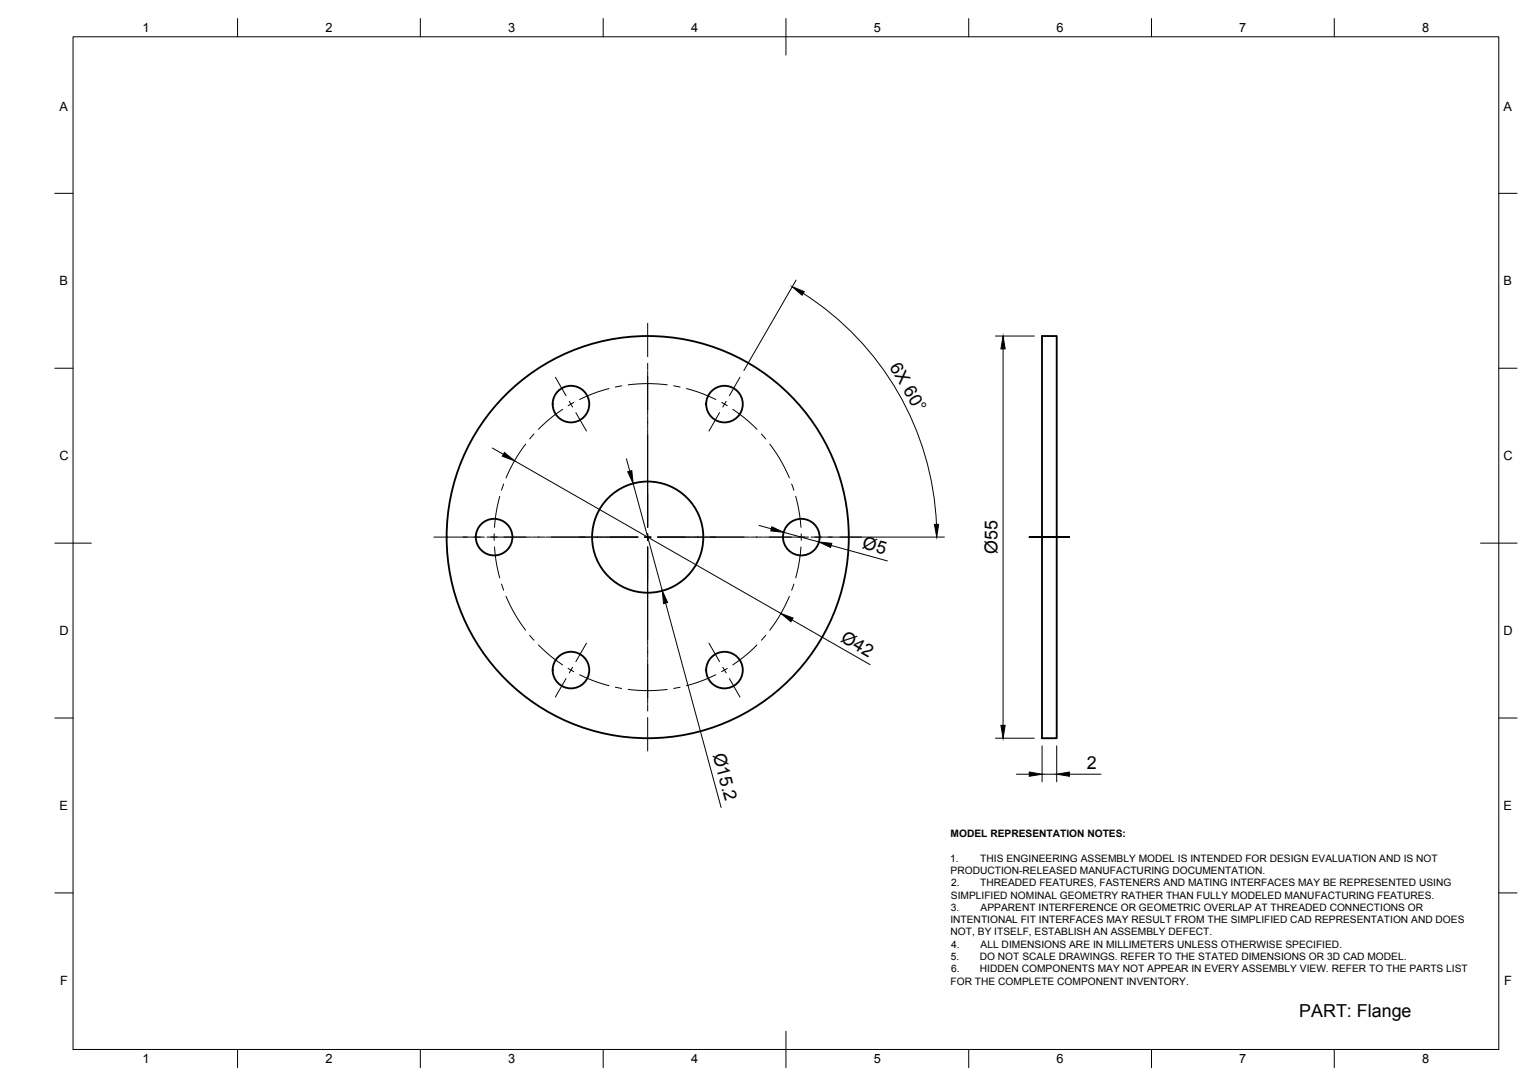
ISO-10303-21;
HEADER;
/* Generated by software containing ST-Developer
 * from STEP Tools, Inc. (www.steptools.com) 
 */

FILE_DESCRIPTION(
/* description */ ('STEP AP214'),
/* implementation_level */ '2;1');

FILE_NAME(
/* name */ 'Flange.step',
/* time_stamp */ '2026-10-05T13:15:56-07:00',
/* author */ (''),
/* organization */ (''),
/* preprocessor_version */ 'ST-DEVELOPER v20.2',
/* originating_system */ 'Autodesk Translation Framework v15.15.0.0',
/* authorisation */ '');

FILE_SCHEMA (('AUTOMOTIVE_DESIGN { 1 0 10303 214 3 1 1 }'));
ENDSEC;

DATA;
#10=MECHANICAL_DESIGN_GEOMETRIC_PRESENTATION_REPRESENTATION('',(#1352),#37881);
#1328=SHAPE_REPRESENTATION_RELATIONSHIP('SRR','None',#37961,#1340);
#1340=ADVANCED_BREP_SHAPE_REPRESENTATION('',(#1364),#37876);
#1352=STYLED_ITEM('',(#38023),#1364);
#1364=MANIFOLD_SOLID_BREP('Body1',#10826);
#1447=FACE_BOUND('',#2815,.T.);
#1448=FACE_BOUND('',#2816,.T.);
#1449=FACE_BOUND('',#2817,.T.);
#1450=FACE_BOUND('',#2818,.T.);
#1451=FACE_BOUND('',#2819,.T.);
#1452=FACE_BOUND('',#2820,.T.);
#1453=FACE_BOUND('',#2821,.T.);
#1454=FACE_BOUND('',#2823,.T.);
#1455=FACE_BOUND('',#2824,.T.);
#1456=FACE_BOUND('',#2825,.T.);
#1457=FACE_BOUND('',#2826,.T.);
#1458=FACE_BOUND('',#2827,.T.);
#1459=FACE_BOUND('',#2828,.T.);
#1460=FACE_BOUND('',#2829,.T.);
#1533=PLANE('',#11792);
#1534=PLANE('',#11793);
#2127=FACE_OUTER_BOUND('',#2806,.T.);
#2128=FACE_OUTER_BOUND('',#2807,.T.);
#2129=FACE_OUTER_BOUND('',#2808,.T.);
#2130=FACE_OUTER_BOUND('',#2809,.T.);
#2131=FACE_OUTER_BOUND('',#2810,.T.);
#2132=FACE_OUTER_BOUND('',#2811,.T.);
#2133=FACE_OUTER_BOUND('',#2812,.T.);
#2134=FACE_OUTER_BOUND('',#2813,.T.);
#2135=FACE_OUTER_BOUND('',#2814,.T.);
#2136=FACE_OUTER_BOUND('',#2822,.T.);
#2806=EDGE_LOOP('',(#9821,#9822,#9823,#9824));
#2807=EDGE_LOOP('',(#9825,#9826,#9827,#9828));
#2808=EDGE_LOOP('',(#9829,#9830,#9831,#9832));
#2809=EDGE_LOOP('',(#9833,#9834,#9835,#9836));
#2810=EDGE_LOOP('',(#9837,#9838,#9839,#9840));
#2811=EDGE_LOOP('',(#9841,#9842,#9843,#9844));
#2812=EDGE_LOOP('',(#9845,#9846,#9847,#9848));
#2813=EDGE_LOOP('',(#9849,#9850,#9851,#9852));
#2814=EDGE_LOOP('',(#9853));
#2815=EDGE_LOOP('',(#9854));
#2816=EDGE_LOOP('',(#9855));
#2817=EDGE_LOOP('',(#9856));
#2818=EDGE_LOOP('',(#9857));
#2819=EDGE_LOOP('',(#9858));
#2820=EDGE_LOOP('',(#9859));
#2821=EDGE_LOOP('',(#9860));
#2822=EDGE_LOOP('',(#9861));
#2823=EDGE_LOOP('',(#9862));
#2824=EDGE_LOOP('',(#9863));
#2825=EDGE_LOOP('',(#9864));
#2826=EDGE_LOOP('',(#9865));
#2827=EDGE_LOOP('',(#9866));
#2828=EDGE_LOOP('',(#9867));
#2829=EDGE_LOOP('',(#9868));
#3098=LINE('',#37593,#3399);
#3099=LINE('',#37599,#3400);
#3100=LINE('',#37605,#3401);
#3101=LINE('',#37611,#3402);
#3102=LINE('',#37617,#3403);
#3103=LINE('',#37623,#3404);
#3104=LINE('',#37629,#3405);
#3105=LINE('',#37635,#3406);
#3399=VECTOR('',#13729,2.5);
#3400=VECTOR('',#13736,2.5);
#3401=VECTOR('',#13743,2.5);
#3402=VECTOR('',#13750,2.5);
#3403=VECTOR('',#13757,2.5);
#3404=VECTOR('',#13764,2.5);
#3405=VECTOR('',#13771,7.6);
#3406=VECTOR('',#13778,27.5);
#3968=CIRCLE('',#11769,2.5);
#3969=CIRCLE('',#11770,2.5);
#3970=CIRCLE('',#11772,2.5);
#3971=CIRCLE('',#11773,2.5);
#3972=CIRCLE('',#11775,2.5);
#3973=CIRCLE('',#11776,2.5);
#3974=CIRCLE('',#11778,2.5);
#3975=CIRCLE('',#11779,2.5);
#3976=CIRCLE('',#11781,2.5);
#3977=CIRCLE('',#11782,2.5);
#3978=CIRCLE('',#11784,2.5);
#3979=CIRCLE('',#11785,2.5);
#3980=CIRCLE('',#11787,7.6);
#3981=CIRCLE('',#11788,7.6);
#3982=CIRCLE('',#11790,27.5);
#3983=CIRCLE('',#11791,27.5);
#5004=VERTEX_POINT('',#37590);
#5005=VERTEX_POINT('',#37592);
#5006=VERTEX_POINT('',#37596);
#5007=VERTEX_POINT('',#37598);
#5008=VERTEX_POINT('',#37602);
#5009=VERTEX_POINT('',#37604);
#5010=VERTEX_POINT('',#37608);
#5011=VERTEX_POINT('',#37610);
#5012=VERTEX_POINT('',#37614);
#5013=VERTEX_POINT('',#37616);
#5014=VERTEX_POINT('',#37620);
#5015=VERTEX_POINT('',#37622);
#5016=VERTEX_POINT('',#37626);
#5017=VERTEX_POINT('',#37628);
#5018=VERTEX_POINT('',#37632);
#5019=VERTEX_POINT('',#37634);
#6621=EDGE_CURVE('',#5004,#5004,#3968,.T.);
#6622=EDGE_CURVE('',#5004,#5005,#3098,.T.);
#6623=EDGE_CURVE('',#5005,#5005,#3969,.T.);
#6624=EDGE_CURVE('',#5006,#5006,#3970,.T.);
#6625=EDGE_CURVE('',#5006,#5007,#3099,.T.);
#6626=EDGE_CURVE('',#5007,#5007,#3971,.T.);
#6627=EDGE_CURVE('',#5008,#5008,#3972,.T.);
#6628=EDGE_CURVE('',#5008,#5009,#3100,.T.);
#6629=EDGE_CURVE('',#5009,#5009,#3973,.T.);
#6630=EDGE_CURVE('',#5010,#5010,#3974,.T.);
#6631=EDGE_CURVE('',#5010,#5011,#3101,.T.);
#6632=EDGE_CURVE('',#5011,#5011,#3975,.T.);
#6633=EDGE_CURVE('',#5012,#5012,#3976,.T.);
#6634=EDGE_CURVE('',#5012,#5013,#3102,.T.);
#6635=EDGE_CURVE('',#5013,#5013,#3977,.T.);
#6636=EDGE_CURVE('',#5014,#5014,#3978,.T.);
#6637=EDGE_CURVE('',#5014,#5015,#3103,.T.);
#6638=EDGE_CURVE('',#5015,#5015,#3979,.T.);
#6639=EDGE_CURVE('',#5016,#5016,#3980,.T.);
#6640=EDGE_CURVE('',#5016,#5017,#3104,.T.);
#6641=EDGE_CURVE('',#5017,#5017,#3981,.T.);
#6642=EDGE_CURVE('',#5018,#5018,#3982,.T.);
#6643=EDGE_CURVE('',#5018,#5019,#3105,.T.);
#6644=EDGE_CURVE('',#5019,#5019,#3983,.T.);
#9821=ORIENTED_EDGE('',*,*,#6621,.T.);
#9822=ORIENTED_EDGE('',*,*,#6622,.T.);
#9823=ORIENTED_EDGE('',*,*,#6623,.F.);
#9824=ORIENTED_EDGE('',*,*,#6622,.F.);
#9825=ORIENTED_EDGE('',*,*,#6624,.T.);
#9826=ORIENTED_EDGE('',*,*,#6625,.T.);
#9827=ORIENTED_EDGE('',*,*,#6626,.F.);
#9828=ORIENTED_EDGE('',*,*,#6625,.F.);
#9829=ORIENTED_EDGE('',*,*,#6627,.T.);
#9830=ORIENTED_EDGE('',*,*,#6628,.T.);
#9831=ORIENTED_EDGE('',*,*,#6629,.F.);
#9832=ORIENTED_EDGE('',*,*,#6628,.F.);
#9833=ORIENTED_EDGE('',*,*,#6630,.T.);
#9834=ORIENTED_EDGE('',*,*,#6631,.T.);
#9835=ORIENTED_EDGE('',*,*,#6632,.F.);
#9836=ORIENTED_EDGE('',*,*,#6631,.F.);
#9837=ORIENTED_EDGE('',*,*,#6633,.T.);
#9838=ORIENTED_EDGE('',*,*,#6634,.T.);
#9839=ORIENTED_EDGE('',*,*,#6635,.F.);
#9840=ORIENTED_EDGE('',*,*,#6634,.F.);
#9841=ORIENTED_EDGE('',*,*,#6636,.T.);
#9842=ORIENTED_EDGE('',*,*,#6637,.T.);
#9843=ORIENTED_EDGE('',*,*,#6638,.F.);
#9844=ORIENTED_EDGE('',*,*,#6637,.F.);
#9845=ORIENTED_EDGE('',*,*,#6639,.T.);
#9846=ORIENTED_EDGE('',*,*,#6640,.T.);
#9847=ORIENTED_EDGE('',*,*,#6641,.F.);
#9848=ORIENTED_EDGE('',*,*,#6640,.F.);
#9849=ORIENTED_EDGE('',*,*,#6642,.T.);
#9850=ORIENTED_EDGE('',*,*,#6643,.T.);
#9851=ORIENTED_EDGE('',*,*,#6644,.F.);
#9852=ORIENTED_EDGE('',*,*,#6643,.F.);
#9853=ORIENTED_EDGE('',*,*,#6644,.T.);
#9854=ORIENTED_EDGE('',*,*,#6639,.F.);
#9855=ORIENTED_EDGE('',*,*,#6633,.F.);
#9856=ORIENTED_EDGE('',*,*,#6627,.F.);
#9857=ORIENTED_EDGE('',*,*,#6621,.F.);
#9858=ORIENTED_EDGE('',*,*,#6624,.F.);
#9859=ORIENTED_EDGE('',*,*,#6630,.F.);
#9860=ORIENTED_EDGE('',*,*,#6636,.F.);
#9861=ORIENTED_EDGE('',*,*,#6642,.F.);
#9862=ORIENTED_EDGE('',*,*,#6641,.T.);
#9863=ORIENTED_EDGE('',*,*,#6638,.T.);
#9864=ORIENTED_EDGE('',*,*,#6635,.T.);
#9865=ORIENTED_EDGE('',*,*,#6632,.T.);
#9866=ORIENTED_EDGE('',*,*,#6629,.T.);
#9867=ORIENTED_EDGE('',*,*,#6626,.T.);
#9868=ORIENTED_EDGE('',*,*,#6623,.T.);
#10197=CYLINDRICAL_SURFACE('',#11768,2.5);
#10198=CYLINDRICAL_SURFACE('',#11771,2.5);
#10199=CYLINDRICAL_SURFACE('',#11774,2.5);
#10200=CYLINDRICAL_SURFACE('',#11777,2.5);
#10201=CYLINDRICAL_SURFACE('',#11780,2.5);
#10202=CYLINDRICAL_SURFACE('',#11783,2.5);
#10203=CYLINDRICAL_SURFACE('',#11786,7.6);
#10204=CYLINDRICAL_SURFACE('',#11789,27.5);
#10772=ADVANCED_FACE('',(#2127),#10197,.F.);
#10773=ADVANCED_FACE('',(#2128),#10198,.F.);
#10774=ADVANCED_FACE('',(#2129),#10199,.F.);
#10775=ADVANCED_FACE('',(#2130),#10200,.F.);
#10776=ADVANCED_FACE('',(#2131),#10201,.F.);
#10777=ADVANCED_FACE('',(#2132),#10202,.F.);
#10778=ADVANCED_FACE('',(#2133),#10203,.F.);
#10779=ADVANCED_FACE('',(#2134),#10204,.T.);
#10780=ADVANCED_FACE('',(#2135,#1447,#1448,#1449,#1450,#1451,#1452,#1453),
#1533,.T.);
#10781=ADVANCED_FACE('',(#2136,#1454,#1455,#1456,#1457,#1458,#1459,#1460),
#1534,.F.);
#10826=CLOSED_SHELL('',(#10772,#10773,#10774,#10775,#10776,#10777,#10778,
#10779,#10780,#10781));
#11767=AXIS2_PLACEMENT_3D('',#37588,#13723,#13724);
#11768=AXIS2_PLACEMENT_3D('',#37589,#13725,#13726);
#11769=AXIS2_PLACEMENT_3D('',#37591,#13727,#13728);
#11770=AXIS2_PLACEMENT_3D('',#37594,#13730,#13731);
#11771=AXIS2_PLACEMENT_3D('',#37595,#13732,#13733);
#11772=AXIS2_PLACEMENT_3D('',#37597,#13734,#13735);
#11773=AXIS2_PLACEMENT_3D('',#37600,#13737,#13738);
#11774=AXIS2_PLACEMENT_3D('',#37601,#13739,#13740);
#11775=AXIS2_PLACEMENT_3D('',#37603,#13741,#13742);
#11776=AXIS2_PLACEMENT_3D('',#37606,#13744,#13745);
#11777=AXIS2_PLACEMENT_3D('',#37607,#13746,#13747);
#11778=AXIS2_PLACEMENT_3D('',#37609,#13748,#13749);
#11779=AXIS2_PLACEMENT_3D('',#37612,#13751,#13752);
#11780=AXIS2_PLACEMENT_3D('',#37613,#13753,#13754);
#11781=AXIS2_PLACEMENT_3D('',#37615,#13755,#13756);
#11782=AXIS2_PLACEMENT_3D('',#37618,#13758,#13759);
#11783=AXIS2_PLACEMENT_3D('',#37619,#13760,#13761);
#11784=AXIS2_PLACEMENT_3D('',#37621,#13762,#13763);
#11785=AXIS2_PLACEMENT_3D('',#37624,#13765,#13766);
#11786=AXIS2_PLACEMENT_3D('',#37625,#13767,#13768);
#11787=AXIS2_PLACEMENT_3D('',#37627,#13769,#13770);
#11788=AXIS2_PLACEMENT_3D('',#37630,#13772,#13773);
#11789=AXIS2_PLACEMENT_3D('',#37631,#13774,#13775);
#11790=AXIS2_PLACEMENT_3D('',#37633,#13776,#13777);
#11791=AXIS2_PLACEMENT_3D('',#37636,#13779,#13780);
#11792=AXIS2_PLACEMENT_3D('',#37637,#13781,#13782);
#11793=AXIS2_PLACEMENT_3D('',#37638,#13783,#13784);
#13723=DIRECTION('axis',(0.,0.,1.));
#13724=DIRECTION('refdir',(1.,0.,0.));
#13725=DIRECTION('center_axis',(-2.36658271566304E-30,1.04667633103075E-31,
-1.));
#13726=DIRECTION('ref_axis',(-1.,-2.47704611391098E-61,2.36658271566304E-30));
#13727=DIRECTION('center_axis',(2.36658271566304E-30,-1.04667633103075E-31,
1.));
#13728=DIRECTION('ref_axis',(1.,2.47704611391098E-61,-2.36658271566304E-30));
#13729=DIRECTION('',(-2.36658271566304E-30,1.04667633103075E-31,-1.));
#13730=DIRECTION('center_axis',(2.36658271566304E-30,-1.04667633103075E-31,
1.));
#13731=DIRECTION('ref_axis',(1.,2.47704611391098E-61,-2.36658271566304E-30));
#13732=DIRECTION('center_axis',(-2.36658271566304E-30,1.04667633103075E-31,
-1.));
#13733=DIRECTION('ref_axis',(-1.,-2.47704611391098E-61,2.36658271566304E-30));
#13734=DIRECTION('center_axis',(2.36658271566304E-30,-1.04667633103075E-31,
1.));
#13735=DIRECTION('ref_axis',(1.,2.47704611391098E-61,-2.36658271566304E-30));
#13736=DIRECTION('',(-2.36658271566304E-30,1.04667633103075E-31,-1.));
#13737=DIRECTION('center_axis',(2.36658271566304E-30,-1.04667633103075E-31,
1.));
#13738=DIRECTION('ref_axis',(1.,2.47704611391098E-61,-2.36658271566304E-30));
#13739=DIRECTION('center_axis',(-2.36658271566304E-30,1.04667633103075E-31,
-1.));
#13740=DIRECTION('ref_axis',(-1.,-2.47704611391098E-61,2.36658271566304E-30));
#13741=DIRECTION('center_axis',(2.36658271566304E-30,-1.04667633103075E-31,
1.));
#13742=DIRECTION('ref_axis',(1.,2.47704611391098E-61,-2.36658271566304E-30));
#13743=DIRECTION('',(-2.36658271566304E-30,1.04667633103075E-31,-1.));
#13744=DIRECTION('center_axis',(2.36658271566304E-30,-1.04667633103075E-31,
1.));
#13745=DIRECTION('ref_axis',(1.,2.47704611391098E-61,-2.36658271566304E-30));
#13746=DIRECTION('center_axis',(-2.36658271566304E-30,1.04667633103075E-31,
-1.));
#13747=DIRECTION('ref_axis',(-1.,-2.47704611391098E-61,2.36658271566304E-30));
#13748=DIRECTION('center_axis',(2.36658271566304E-30,-1.04667633103075E-31,
1.));
#13749=DIRECTION('ref_axis',(1.,2.47704611391098E-61,-2.36658271566304E-30));
#13750=DIRECTION('',(-2.36658271566304E-30,1.04667633103075E-31,-1.));
#13751=DIRECTION('center_axis',(2.36658271566304E-30,-1.04667633103075E-31,
1.));
#13752=DIRECTION('ref_axis',(1.,2.47704611391098E-61,-2.36658271566304E-30));
#13753=DIRECTION('center_axis',(-2.36658271566304E-30,1.04667633103075E-31,
-1.));
#13754=DIRECTION('ref_axis',(-1.,-2.47704611391098E-61,2.36658271566304E-30));
#13755=DIRECTION('center_axis',(2.36658271566304E-30,-1.04667633103075E-31,
1.));
#13756=DIRECTION('ref_axis',(1.,2.47704611391098E-61,-2.36658271566304E-30));
#13757=DIRECTION('',(-2.36658271566304E-30,1.04667633103075E-31,-1.));
#13758=DIRECTION('center_axis',(2.36658271566304E-30,-1.04667633103075E-31,
1.));
#13759=DIRECTION('ref_axis',(1.,2.47704611391098E-61,-2.36658271566304E-30));
#13760=DIRECTION('center_axis',(-2.36658271566304E-30,1.04667633103075E-31,
-1.));
#13761=DIRECTION('ref_axis',(-1.,-2.47704611391098E-61,2.36658271566304E-30));
#13762=DIRECTION('center_axis',(2.36658271566304E-30,-1.04667633103075E-31,
1.));
#13763=DIRECTION('ref_axis',(1.,2.47704611391098E-61,-2.36658271566304E-30));
#13764=DIRECTION('',(-2.36658271566304E-30,1.04667633103075E-31,-1.));
#13765=DIRECTION('center_axis',(2.36658271566304E-30,-1.04667633103075E-31,
1.));
#13766=DIRECTION('ref_axis',(1.,2.47704611391098E-61,-2.36658271566304E-30));
#13767=DIRECTION('center_axis',(-2.36658271566304E-30,1.04667633103075E-31,
-1.));
#13768=DIRECTION('ref_axis',(-1.,-2.47704611391098E-61,2.36658271566304E-30));
#13769=DIRECTION('center_axis',(2.36658271566304E-30,-1.04667633103075E-31,
1.));
#13770=DIRECTION('ref_axis',(1.,2.47704611391098E-61,-2.36658271566304E-30));
#13771=DIRECTION('',(-2.36658271566304E-30,1.04667633103075E-31,-1.));
#13772=DIRECTION('center_axis',(2.36658271566304E-30,-1.04667633103075E-31,
1.));
#13773=DIRECTION('ref_axis',(1.,2.47704611391098E-61,-2.36658271566304E-30));
#13774=DIRECTION('center_axis',(-2.36658271566304E-30,1.04667633103075E-31,
-1.));
#13775=DIRECTION('ref_axis',(-1.,-2.47704611391098E-61,2.36658271566304E-30));
#13776=DIRECTION('center_axis',(2.36658271566304E-30,-1.04667633103075E-31,
1.));
#13777=DIRECTION('ref_axis',(1.,2.47704611391098E-61,-2.36658271566304E-30));
#13778=DIRECTION('',(2.36658271566304E-30,-1.04667633103075E-31,1.));
#13779=DIRECTION('center_axis',(2.36658271566304E-30,-1.04667633103075E-31,
1.));
#13780=DIRECTION('ref_axis',(1.,2.47704611391098E-61,-2.36658271566304E-30));
#13781=DIRECTION('center_axis',(-2.36658271566304E-30,-1.04667633103075E-31,
1.));
#13782=DIRECTION('ref_axis',(1.,0.,2.36658271566304E-30));
#13783=DIRECTION('center_axis',(-2.36658271566304E-30,-1.04667633103075E-31,
1.));
#13784=DIRECTION('ref_axis',(1.,0.,2.36658271566304E-30));
#37588=CARTESIAN_POINT('',(0.,0.,0.));
#37589=CARTESIAN_POINT('Origin',(-18.1865334794732,10.5,1.));
#37590=CARTESIAN_POINT('',(-15.6865334794732,10.5,1.));
#37591=CARTESIAN_POINT('Origin',(-18.1865334794732,10.5,1.));
#37592=CARTESIAN_POINT('',(-15.6865334794732,10.5,-1.));
#37593=CARTESIAN_POINT('',(-15.6865334794732,10.5,1.));
#37594=CARTESIAN_POINT('Origin',(-18.1865334794732,10.5,-1.));
#37595=CARTESIAN_POINT('Origin',(-18.1865334794732,-10.5,1.));
#37596=CARTESIAN_POINT('',(-15.6865334794732,-10.5,1.));
#37597=CARTESIAN_POINT('Origin',(-18.1865334794732,-10.5,1.));
#37598=CARTESIAN_POINT('',(-15.6865334794732,-10.5,-1.));
#37599=CARTESIAN_POINT('',(-15.6865334794732,-10.5,1.));
#37600=CARTESIAN_POINT('Origin',(-18.1865334794732,-10.5,-1.));
#37601=CARTESIAN_POINT('Origin',(6.93889390390723E-15,-21.,1.));
#37602=CARTESIAN_POINT('',(2.50000000000001,-21.,1.));
#37603=CARTESIAN_POINT('Origin',(6.93889390390723E-15,-21.,1.));
#37604=CARTESIAN_POINT('',(2.50000000000001,-21.,-1.));
#37605=CARTESIAN_POINT('',(2.50000000000001,-21.,1.));
#37606=CARTESIAN_POINT('Origin',(6.93889390390723E-15,-21.,-1.));
#37607=CARTESIAN_POINT('Origin',(18.1865334794732,-10.5,1.));
#37608=CARTESIAN_POINT('',(20.6865334794732,-10.5,1.));
#37609=CARTESIAN_POINT('Origin',(18.1865334794732,-10.5,1.));
#37610=CARTESIAN_POINT('',(20.6865334794732,-10.5,-0.99999999999998));
#37611=CARTESIAN_POINT('',(20.6865334794732,-10.5,1.));
#37612=CARTESIAN_POINT('Origin',(18.1865334794732,-10.5,-0.99999999999998));
#37613=CARTESIAN_POINT('Origin',(18.1865334794732,10.5,1.));
#37614=CARTESIAN_POINT('',(20.6865334794732,10.5,1.));
#37615=CARTESIAN_POINT('Origin',(18.1865334794732,10.5,1.));
#37616=CARTESIAN_POINT('',(20.6865334794732,10.5,-0.99999999999998));
#37617=CARTESIAN_POINT('',(20.6865334794732,10.5,1.));
#37618=CARTESIAN_POINT('Origin',(18.1865334794732,10.5,-0.99999999999998));
#37619=CARTESIAN_POINT('Origin',(0.,21.,1.));
#37620=CARTESIAN_POINT('',(2.5,21.,1.));
#37621=CARTESIAN_POINT('Origin',(0.,21.,1.));
#37622=CARTESIAN_POINT('',(2.5,21.,-1.));
#37623=CARTESIAN_POINT('',(2.5,21.,1.));
#37624=CARTESIAN_POINT('Origin',(0.,21.,-1.));
#37625=CARTESIAN_POINT('Origin',(0.,0.,1.));
#37626=CARTESIAN_POINT('',(7.6,-9.30731567351989E-16,1.));
#37627=CARTESIAN_POINT('Origin',(0.,0.,1.));
#37628=CARTESIAN_POINT('',(7.6,-9.30731567351988E-16,-1.));
#37629=CARTESIAN_POINT('',(7.6,-9.30731567351989E-16,1.));
#37630=CARTESIAN_POINT('Origin',(0.,0.,-1.));
#37631=CARTESIAN_POINT('Origin',(0.,0.,1.));
#37632=CARTESIAN_POINT('',(27.5,-3.36777869765522E-15,-1.));
#37633=CARTESIAN_POINT('Origin',(0.,0.,-1.));
#37634=CARTESIAN_POINT('',(27.5,-3.36777869765522E-15,1.));
#37635=CARTESIAN_POINT('',(27.5,-3.36777869765522E-15,1.));
#37636=CARTESIAN_POINT('Origin',(0.,0.,1.));
#37637=CARTESIAN_POINT('Origin',(0.,0.,1.));
#37638=CARTESIAN_POINT('Origin',(0.,0.,-1.));
#37862=UNCERTAINTY_MEASURE_WITH_UNIT(LENGTH_MEASURE(0.01),#37882,
'DISTANCE_ACCURACY_VALUE',
'Maximum model space distance between geometric entities at asserted c
onnectivities');
#37867=UNCERTAINTY_MEASURE_WITH_UNIT(LENGTH_MEASURE(0.01),#37882,
'DISTANCE_ACCURACY_VALUE',
'Maximum model space distance between geometric entities at asserted c
onnectivities');
#37876=(
GEOMETRIC_REPRESENTATION_CONTEXT(3)
GLOBAL_UNCERTAINTY_ASSIGNED_CONTEXT((#37862))
GLOBAL_UNIT_ASSIGNED_CONTEXT((#37882,#37884,#37885))
REPRESENTATION_CONTEXT('','3D')
);
#37881=(
GEOMETRIC_REPRESENTATION_CONTEXT(3)
GLOBAL_UNCERTAINTY_ASSIGNED_CONTEXT((#37867))
GLOBAL_UNIT_ASSIGNED_CONTEXT((#37882,#37884,#37885))
REPRESENTATION_CONTEXT('','3D')
);
#37882=(
LENGTH_UNIT()
NAMED_UNIT(*)
SI_UNIT(.MILLI.,.METRE.)
);
#37884=(
NAMED_UNIT(*)
PLANE_ANGLE_UNIT()
SI_UNIT($,.RADIAN.)
);
#37885=(
NAMED_UNIT(*)
SI_UNIT($,.STERADIAN.)
SOLID_ANGLE_UNIT()
);
#37894=SHAPE_DEFINITION_REPRESENTATION(#37907,#37961);
#37907=PRODUCT_DEFINITION_SHAPE('',$,#37975);
#37961=SHAPE_REPRESENTATION('',(#11767),#37876);
#37966=PRODUCT_DEFINITION_CONTEXT('part definition',#38007,'design');
#37975=PRODUCT_DEFINITION('PS04','Flange',#37988,#37966);
#37988=PRODUCT_DEFINITION_FORMATION('',$,#38017);
#38007=APPLICATION_CONTEXT(
'Core Data for Automotive Mechanical Design Process');
#38008=PRODUCT_CONTEXT('part definition',#38007,'mechanical');
#38017=PRODUCT('PS04','Flange',$,(#38008));
#38023=PRESENTATION_STYLE_ASSIGNMENT((#38025));
#38025=SURFACE_STYLE_USAGE(.BOTH.,#38027);
#38027=SURFACE_SIDE_STYLE('',(#38029));
#38029=SURFACE_STYLE_FILL_AREA(#38031);
#38031=FILL_AREA_STYLE('Opaque(202,209,238)',(#38033));
#38033=FILL_AREA_STYLE_COLOUR('Opaque(202,209,238)',#38035);
#38035=COLOUR_RGB('Opaque(202,209,238)', 0.66274510, 0.83137255, 0.94901961);
ENDSEC;
END-ISO-10303-21;
